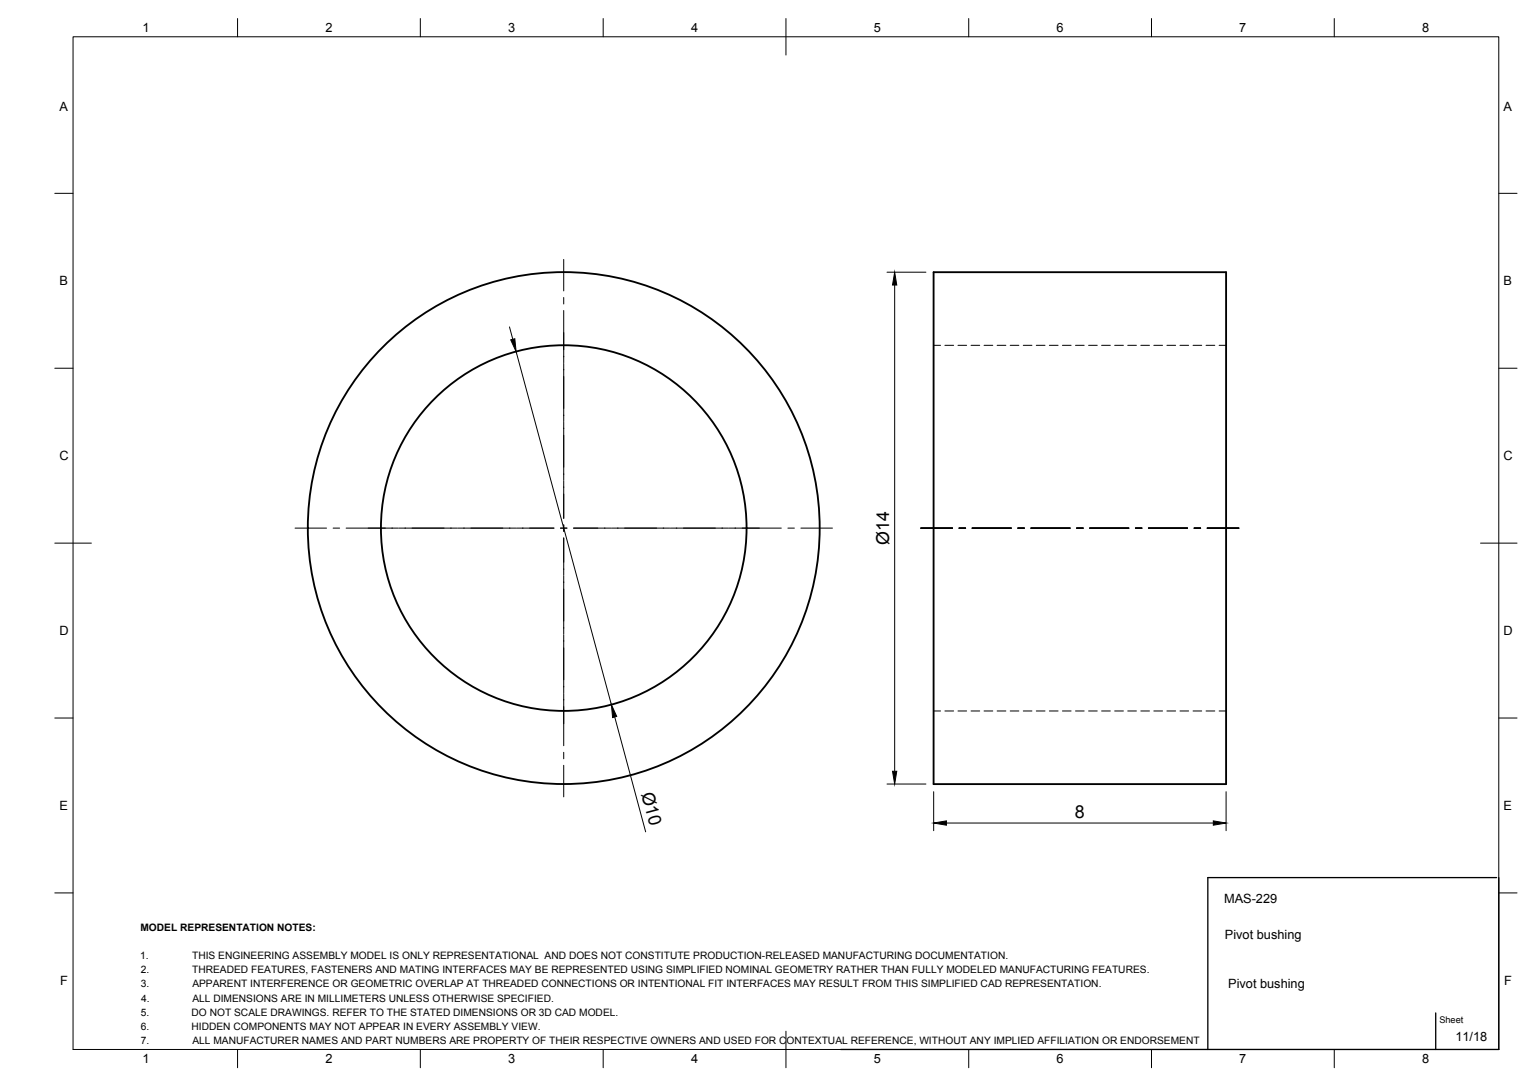
ISO-10303-21;
HEADER;
/* Generated by software containing ST-Developer
 * from STEP Tools, Inc. (www.steptools.com) 
 */

FILE_DESCRIPTION(
/* description */ ('Independently dimensioned six-bar single-leg walking-linkage demonstr
ator. Whole-mm20 crank,60 upper rocker,80/120 ternary coupler,120 lowe
r rocker,140 knee pitch and260 toe reach; ground pivots0/0,60/0,40/60.
 Seven native revolutes close both loops. Four reused native library f
amilies, fully retained shared pins and layered real spacer stacks, bo
nded rubber toe. Benchtop reference mechanism; no complete vehicle, lo
ad, gait stability, adhesive, weld, fit or life rating.'),
/* implementation_level */ '2;1');

FILE_NAME(
/* name */ 'Pivot bushing.step',
/* time_stamp */ '2026-11-09T20:33:14-08:00',
/* author */ (''),
/* organization */ (''),
/* preprocessor_version */ 'ST-DEVELOPER v20.2',
/* originating_system */ 'Autodesk Translation Framework v15.17.0.0',
/* authorisation */ '');

FILE_SCHEMA (('AUTOMOTIVE_DESIGN { 1 0 10303 214 3 1 1 }'));
ENDSEC;

DATA;
#10=MECHANICAL_DESIGN_GEOMETRIC_PRESENTATION_REPRESENTATION('',(#263),#4048);
#227=SHAPE_REPRESENTATION_RELATIONSHIP('SRR','None',#4151,#245);
#245=ADVANCED_BREP_SHAPE_REPRESENTATION('',(#281),#4038);
#263=STYLED_ITEM('',(#4250),#281);
#281=MANIFOLD_SOLID_BREP('Body1',#2152);
#327=FACE_BOUND('',#645,.T.);
#328=FACE_BOUND('',#647,.T.);
#384=PLANE('',#2500);
#385=PLANE('',#2501);
#480=FACE_OUTER_BOUND('',#642,.T.);
#481=FACE_OUTER_BOUND('',#643,.T.);
#482=FACE_OUTER_BOUND('',#644,.T.);
#483=FACE_OUTER_BOUND('',#646,.T.);
#642=EDGE_LOOP('',(#1779,#1780,#1781,#1782));
#643=EDGE_LOOP('',(#1783,#1784,#1785,#1786));
#644=EDGE_LOOP('',(#1787));
#645=EDGE_LOOP('',(#1788));
#646=EDGE_LOOP('',(#1789));
#647=EDGE_LOOP('',(#1790));
#813=LINE('',#3740,#938);
#814=LINE('',#3746,#939);
#938=VECTOR('',#3030,5.);
#939=VECTOR('',#3037,7.);
#1032=CIRCLE('',#2495,5.);
#1033=CIRCLE('',#2496,5.);
#1034=CIRCLE('',#2498,7.);
#1035=CIRCLE('',#2499,7.);
#1186=VERTEX_POINT('',#3737);
#1187=VERTEX_POINT('',#3739);
#1188=VERTEX_POINT('',#3743);
#1189=VERTEX_POINT('',#3745);
#1393=EDGE_CURVE('',#1186,#1186,#1032,.T.);
#1394=EDGE_CURVE('',#1186,#1187,#813,.T.);
#1395=EDGE_CURVE('',#1187,#1187,#1033,.T.);
#1396=EDGE_CURVE('',#1188,#1188,#1034,.T.);
#1397=EDGE_CURVE('',#1188,#1189,#814,.T.);
#1398=EDGE_CURVE('',#1189,#1189,#1035,.T.);
#1779=ORIENTED_EDGE('',*,*,#1393,.F.);
#1780=ORIENTED_EDGE('',*,*,#1394,.T.);
#1781=ORIENTED_EDGE('',*,*,#1395,.T.);
#1782=ORIENTED_EDGE('',*,*,#1394,.F.);
#1783=ORIENTED_EDGE('',*,*,#1396,.F.);
#1784=ORIENTED_EDGE('',*,*,#1397,.T.);
#1785=ORIENTED_EDGE('',*,*,#1398,.T.);
#1786=ORIENTED_EDGE('',*,*,#1397,.F.);
#1787=ORIENTED_EDGE('',*,*,#1396,.T.);
#1788=ORIENTED_EDGE('',*,*,#1393,.T.);
#1789=ORIENTED_EDGE('',*,*,#1398,.F.);
#1790=ORIENTED_EDGE('',*,*,#1395,.F.);
#1992=CYLINDRICAL_SURFACE('',#2494,5.);
#1993=CYLINDRICAL_SURFACE('',#2497,7.);
#2083=ADVANCED_FACE('',(#480),#1992,.F.);
#2084=ADVANCED_FACE('',(#481),#1993,.T.);
#2085=ADVANCED_FACE('',(#482,#327),#384,.T.);
#2086=ADVANCED_FACE('',(#483,#328),#385,.F.);
#2152=CLOSED_SHELL('',(#2083,#2084,#2085,#2086));
#2493=AXIS2_PLACEMENT_3D('',#3735,#3024,#3025);
#2494=AXIS2_PLACEMENT_3D('',#3736,#3026,#3027);
#2495=AXIS2_PLACEMENT_3D('',#3738,#3028,#3029);
#2496=AXIS2_PLACEMENT_3D('',#3741,#3031,#3032);
#2497=AXIS2_PLACEMENT_3D('',#3742,#3033,#3034);
#2498=AXIS2_PLACEMENT_3D('',#3744,#3035,#3036);
#2499=AXIS2_PLACEMENT_3D('',#3747,#3038,#3039);
#2500=AXIS2_PLACEMENT_3D('',#3748,#3040,#3041);
#2501=AXIS2_PLACEMENT_3D('',#3749,#3042,#3043);
#3024=DIRECTION('axis',(0.,0.,1.));
#3025=DIRECTION('refdir',(1.,0.,0.));
#3026=DIRECTION('center_axis',(0.,0.,1.));
#3027=DIRECTION('ref_axis',(1.,0.,0.));
#3028=DIRECTION('center_axis',(0.,0.,-1.));
#3029=DIRECTION('ref_axis',(1.,0.,0.));
#3030=DIRECTION('',(0.,0.,-1.));
#3031=DIRECTION('center_axis',(0.,0.,-1.));
#3032=DIRECTION('ref_axis',(1.,0.,0.));
#3033=DIRECTION('center_axis',(0.,0.,1.));
#3034=DIRECTION('ref_axis',(1.,0.,0.));
#3035=DIRECTION('center_axis',(0.,0.,1.));
#3036=DIRECTION('ref_axis',(1.,0.,0.));
#3037=DIRECTION('',(0.,0.,-1.));
#3038=DIRECTION('center_axis',(0.,0.,1.));
#3039=DIRECTION('ref_axis',(1.,0.,0.));
#3040=DIRECTION('center_axis',(0.,0.,1.));
#3041=DIRECTION('ref_axis',(1.,0.,0.));
#3042=DIRECTION('center_axis',(0.,0.,1.));
#3043=DIRECTION('ref_axis',(1.,0.,0.));
#3735=CARTESIAN_POINT('',(0.,0.,0.));
#3736=CARTESIAN_POINT('Origin',(0.,0.,0.));
#3737=CARTESIAN_POINT('',(-5.,-6.12323399573677E-16,8.));
#3738=CARTESIAN_POINT('Origin',(0.,0.,8.));
#3739=CARTESIAN_POINT('',(-5.,-6.12323399573677E-16,0.));
#3740=CARTESIAN_POINT('',(-5.,-6.12323399573677E-16,0.));
#3741=CARTESIAN_POINT('Origin',(0.,0.,0.));
#3742=CARTESIAN_POINT('Origin',(0.,0.,0.));
#3743=CARTESIAN_POINT('',(-7.,-8.57252759403147E-16,8.));
#3744=CARTESIAN_POINT('Origin',(0.,0.,8.));
#3745=CARTESIAN_POINT('',(-7.,-8.57252759403147E-16,0.));
#3746=CARTESIAN_POINT('',(-7.,-8.57252759403147E-16,0.));
#3747=CARTESIAN_POINT('Origin',(0.,0.,0.));
#3748=CARTESIAN_POINT('Origin',(0.,0.,8.));
#3749=CARTESIAN_POINT('Origin',(0.,0.,0.));
#4018=UNCERTAINTY_MEASURE_WITH_UNIT(LENGTH_MEASURE(0.01),#4049,
'DISTANCE_ACCURACY_VALUE',
'Maximum model space distance between geometric entities at asserted c
onnectivities');
#4028=UNCERTAINTY_MEASURE_WITH_UNIT(LENGTH_MEASURE(0.01),#4049,
'DISTANCE_ACCURACY_VALUE',
'Maximum model space distance between geometric entities at asserted c
onnectivities');
#4038=(
GEOMETRIC_REPRESENTATION_CONTEXT(3)
GLOBAL_UNCERTAINTY_ASSIGNED_CONTEXT((#4018))
GLOBAL_UNIT_ASSIGNED_CONTEXT((#4049,#4051,#4052))
REPRESENTATION_CONTEXT('','3D')
);
#4048=(
GEOMETRIC_REPRESENTATION_CONTEXT(3)
GLOBAL_UNCERTAINTY_ASSIGNED_CONTEXT((#4028))
GLOBAL_UNIT_ASSIGNED_CONTEXT((#4049,#4051,#4052))
REPRESENTATION_CONTEXT('','3D')
);
#4049=(
LENGTH_UNIT()
NAMED_UNIT(*)
SI_UNIT(.MILLI.,.METRE.)
);
#4051=(
NAMED_UNIT(*)
PLANE_ANGLE_UNIT()
SI_UNIT($,.RADIAN.)
);
#4052=(
NAMED_UNIT(*)
SI_UNIT($,.STERADIAN.)
SOLID_ANGLE_UNIT()
);
#4062=SHAPE_DEFINITION_REPRESENTATION(#4081,#4151);
#4081=PRODUCT_DEFINITION_SHAPE('',$,#4171);
#4151=SHAPE_REPRESENTATION('',(#2493),#4038);
#4161=PRODUCT_DEFINITION_CONTEXT('part definition',#4220,'design');
#4171=PRODUCT_DEFINITION('Pivot bushing','Pivot bushing',#4190,#4161);
#4190=PRODUCT_DEFINITION_FORMATION('',$,#4231);
#4220=APPLICATION_CONTEXT(
'Core Data for Automotive Mechanical Design Process');
#4221=PRODUCT_CONTEXT('part definition',#4220,'mechanical');
#4231=PRODUCT('Pivot bushing','Pivot bushing',$,(#4221));
#4250=PRESENTATION_STYLE_ASSIGNMENT((#4264));
#4264=SURFACE_STYLE_USAGE(.BOTH.,#4278);
#4278=SURFACE_SIDE_STYLE('',(#4292));
#4292=SURFACE_STYLE_FILL_AREA(#4306);
#4306=FILL_AREA_STYLE('Bearing light gray',(#4320));
#4320=FILL_AREA_STYLE_COLOUR('Bearing light gray',#4334);
#4334=COLOUR_RGB('Bearing light gray',0.725490196078431,0.752941176470588,
0.792156862745098);
ENDSEC;
END-ISO-10303-21;
